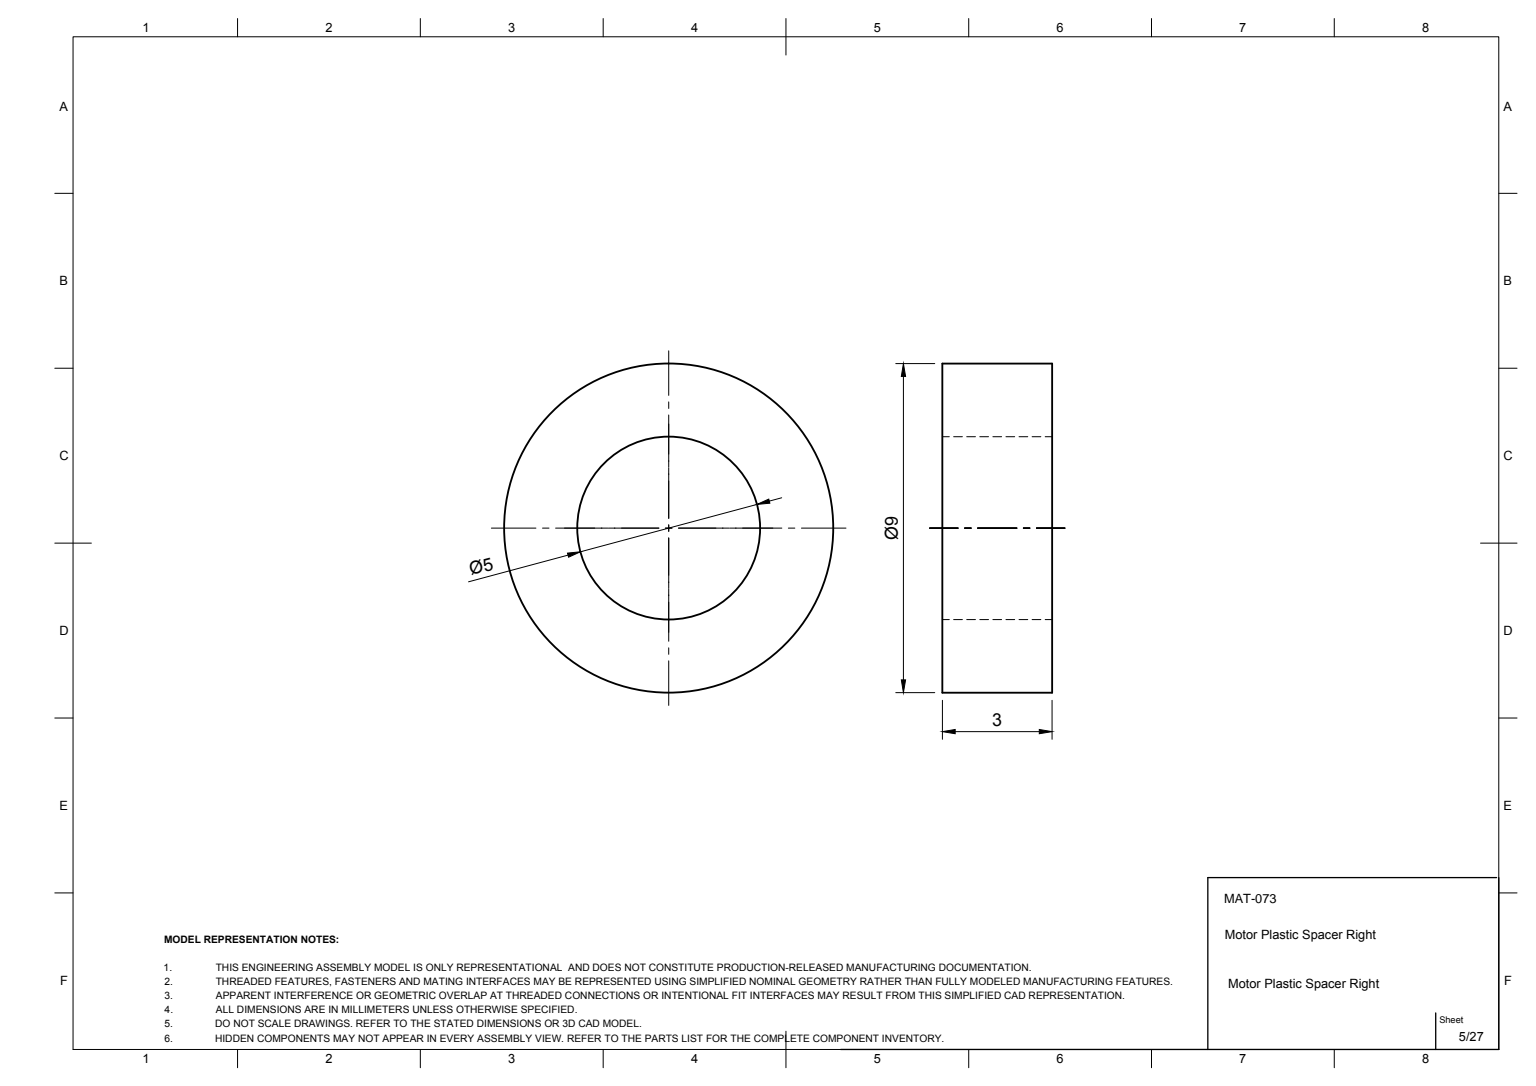
ISO-10303-21;
HEADER;
/* Generated by software containing ST-Developer
 * from STEP Tools, Inc. (www.steptools.com) 
 */

FILE_DESCRIPTION(
/* description */ ('CAx-IF Rec.Pracs.---Representation and Presentation of Product Manufa
cturing Information (PMI)---4.0---2014-10-13'),
/* implementation_level */ '2;1');

FILE_NAME(
/* name */ 'Motor Plastic Spacer Right.step',
/* time_stamp */ '2026-10-24T18:52:33-07:00',
/* author */ (''),
/* organization */ (''),
/* preprocessor_version */ 'ST-DEVELOPER v20.2',
/* originating_system */ 'Autodesk Translation Framework v15.17.0.0',
/* authorisation */ '');

FILE_SCHEMA (('AP242_MANAGED_MODEL_BASED_3D_ENGINEERING_MIM_LF { 1 0 10303 442 2 1 4 }'));
ENDSEC;

DATA;
#10=MECHANICAL_DESIGN_GEOMETRIC_PRESENTATION_REPRESENTATION('',(#416),#34876);
#350=SHAPE_REPRESENTATION_RELATIONSHIP('SRR','None',#34987,#383);
#383=ADVANCED_BREP_SHAPE_REPRESENTATION('',(#449),#34845);
#416=STYLED_ITEM('',(#35161),#449);
#449=MANIFOLD_SOLID_BREP('Motor Plastic Spacer Right',#19556);
#482=FACE_BOUND('',#5883,.T.);
#483=FACE_BOUND('',#5887,.T.);
#606=PLANE('',#20051);
#607=PLANE('',#20058);
#1143=LINE('',#28714,#2742);
#1144=LINE('',#28719,#2743);
#2742=VECTOR('',#22526,0.0025);
#2743=VECTOR('',#22533,0.0045);
#4305=CYLINDRICAL_SURFACE('',#20054,0.0025);
#4306=CYLINDRICAL_SURFACE('',#20056,0.0045);
#4835=FACE_OUTER_BOUND('',#5882,.T.);
#4836=FACE_OUTER_BOUND('',#5884,.T.);
#4837=FACE_OUTER_BOUND('',#5885,.T.);
#4838=FACE_OUTER_BOUND('',#5886,.T.);
#5882=EDGE_LOOP('',(#13034));
#5883=EDGE_LOOP('',(#13035));
#5884=EDGE_LOOP('',(#13036,#13037,#13038,#13039));
#5885=EDGE_LOOP('',(#13040,#13041,#13042,#13043));
#5886=EDGE_LOOP('',(#13044));
#5887=EDGE_LOOP('',(#13045));
#7047=CIRCLE('',#20052,0.00450000000001);
#7048=CIRCLE('',#20053,0.00250000000001);
#7049=CIRCLE('',#20055,0.00250000000001);
#7050=CIRCLE('',#20057,0.00450000000001);
#8149=VERTEX_POINT('',#28708);
#8150=VERTEX_POINT('',#28710);
#8151=VERTEX_POINT('',#28713);
#8152=VERTEX_POINT('',#28717);
#10075=EDGE_CURVE('',#8149,#8149,#7047,.T.);
#10076=EDGE_CURVE('',#8150,#8150,#7048,.T.);
#10077=EDGE_CURVE('',#8150,#8151,#1143,.T.);
#10078=EDGE_CURVE('',#8151,#8151,#7049,.T.);
#10079=EDGE_CURVE('',#8152,#8152,#7050,.T.);
#10080=EDGE_CURVE('',#8152,#8149,#1144,.T.);
#13034=ORIENTED_EDGE('',*,*,#10075,.T.);
#13035=ORIENTED_EDGE('',*,*,#10076,.T.);
#13036=ORIENTED_EDGE('',*,*,#10076,.F.);
#13037=ORIENTED_EDGE('',*,*,#10077,.T.);
#13038=ORIENTED_EDGE('',*,*,#10078,.F.);
#13039=ORIENTED_EDGE('',*,*,#10077,.F.);
#13040=ORIENTED_EDGE('',*,*,#10079,.F.);
#13041=ORIENTED_EDGE('',*,*,#10080,.T.);
#13042=ORIENTED_EDGE('',*,*,#10075,.F.);
#13043=ORIENTED_EDGE('',*,*,#10080,.F.);
#13044=ORIENTED_EDGE('',*,*,#10079,.T.);
#13045=ORIENTED_EDGE('',*,*,#10078,.T.);
#18551=ADVANCED_FACE('',(#4835,#482),#606,.F.);
#18552=ADVANCED_FACE('',(#4836),#4305,.F.);
#18553=ADVANCED_FACE('',(#4837),#4306,.T.);
#18554=ADVANCED_FACE('',(#4838,#483),#607,.T.);
#19556=CLOSED_SHELL('',(#18551,#18552,#18553,#18554));
#20050=AXIS2_PLACEMENT_3D('',#28706,#22516,#22517);
#20051=AXIS2_PLACEMENT_3D('',#28707,#22518,#22519);
#20052=AXIS2_PLACEMENT_3D('',#28709,#22520,#22521);
#20053=AXIS2_PLACEMENT_3D('',#28711,#22522,#22523);
#20054=AXIS2_PLACEMENT_3D('',#28712,#22524,#22525);
#20055=AXIS2_PLACEMENT_3D('',#28715,#22527,#22528);
#20056=AXIS2_PLACEMENT_3D('',#28716,#22529,#22530);
#20057=AXIS2_PLACEMENT_3D('',#28718,#22531,#22532);
#20058=AXIS2_PLACEMENT_3D('',#28720,#22534,#22535);
#22516=DIRECTION('axis',(0.,0.,1.));
#22517=DIRECTION('refdir',(1.,0.,0.));
#22518=DIRECTION('center_axis',(-2.07638679158937E-16,1.,-9.61039042249231E-32));
#22519=DIRECTION('ref_axis',(0.999984788371283,2.07635520636442E-16,-0.00551570721125971));
#22520=DIRECTION('center_axis',(2.07638679158937E-16,-1.,9.61039042249231E-32));
#22521=DIRECTION('ref_axis',(-0.999984788371283,-2.07635520636442E-16,0.00551570721125971));
#22522=DIRECTION('center_axis',(-2.07638679158937E-16,1.,-9.61039042249231E-32));
#22523=DIRECTION('ref_axis',(0.999984788371283,2.07635520636442E-16,-0.00551570721125971));
#22524=DIRECTION('center_axis',(-2.07638679158937E-16,1.,-9.61039042249231E-32));
#22525=DIRECTION('ref_axis',(0.999984788371283,2.07635520636442E-16,-0.00551570721125971));
#22526=DIRECTION('',(-2.07638679158937E-16,1.,-9.61039042249231E-32));
#22527=DIRECTION('center_axis',(2.07638679158937E-16,-1.,9.61039042249231E-32));
#22528=DIRECTION('ref_axis',(0.999984788371283,2.07635520636442E-16,-0.00551570721125971));
#22529=DIRECTION('center_axis',(-2.07638679158937E-16,1.,-9.61039042249231E-32));
#22530=DIRECTION('ref_axis',(-0.999984788371283,-2.07635520636442E-16,0.00551570721125971));
#22531=DIRECTION('center_axis',(-2.07638679158937E-16,1.,-9.61039042249231E-32));
#22532=DIRECTION('ref_axis',(-0.999984788371283,-2.07635520636442E-16,0.00551570721125971));
#22533=DIRECTION('',(2.07638679158937E-16,-1.,9.61039042249231E-32));
#22534=DIRECTION('center_axis',(-2.07638679158937E-16,1.,-9.61039042249231E-32));
#22535=DIRECTION('ref_axis',(0.999984788371283,2.07635520636442E-16,-0.00551570721125971));
#28706=CARTESIAN_POINT('',(0.,0.,0.));
#28707=CARTESIAN_POINT('Origin',(-4.36800060759181E-17,-0.02565,1.40756589985541E-33));
#28708=CARTESIAN_POINT('',(0.00449993154767073,-0.02565000000001,-2.48206824506692E-5));
#28709=CARTESIAN_POINT('Origin',(-4.3680006075916E-17,-0.02565000000001,
1.40756589985638E-33));
#28710=CARTESIAN_POINT('',(-0.00249996197092825,-0.02565000000001,1.37892680281496E-5));
#28711=CARTESIAN_POINT('Origin',(-4.3680006075916E-17,-0.02565000000001,
1.40756589985638E-33));
#28712=CARTESIAN_POINT('Origin',(-4.39914640946565E-17,-0.02415,1.26341004351803E-33));
#28713=CARTESIAN_POINT('',(-0.00249996197092825,-0.02264999999999,1.37892680281496E-5));
#28714=CARTESIAN_POINT('',(-0.00249996197092825,-0.02415,1.37892680281496E-5));
#28715=CARTESIAN_POINT('Origin',(-4.4302922113397E-17,-0.02264999999999,
1.11925418717968E-33));
#28716=CARTESIAN_POINT('Origin',(-4.39914640946565E-17,-0.02415,1.26341004351803E-33));
#28717=CARTESIAN_POINT('',(0.00449993154767073,-0.02264999999999,-2.48206824506692E-5));
#28718=CARTESIAN_POINT('Origin',(-4.4302922113397E-17,-0.02264999999999,
1.11925418717968E-33));
#28719=CARTESIAN_POINT('',(0.00449993154767073,-0.02415,-2.48206824506692E-5));
#28720=CARTESIAN_POINT('Origin',(-4.43029221133949E-17,-0.02265,1.11925418718065E-33));
#34810=UNCERTAINTY_MEASURE_WITH_UNIT(LENGTH_MEASURE(1.E-5),#34877,
'DISTANCE_ACCURACY_VALUE',
'Maximum model space distance between geometric entities at asserted c
onnectivities');
#34841=UNCERTAINTY_MEASURE_WITH_UNIT(LENGTH_MEASURE(1.E-5),#34877,
'DISTANCE_ACCURACY_VALUE',
'Maximum model space distance between geometric entities at asserted c
onnectivities');
#34845=(
GEOMETRIC_REPRESENTATION_CONTEXT(3)
GLOBAL_UNCERTAINTY_ASSIGNED_CONTEXT((#34810))
GLOBAL_UNIT_ASSIGNED_CONTEXT((#34877,#34878,#34879))
REPRESENTATION_CONTEXT('','3D')
);
#34876=(
GEOMETRIC_REPRESENTATION_CONTEXT(3)
GLOBAL_UNCERTAINTY_ASSIGNED_CONTEXT((#34841))
GLOBAL_UNIT_ASSIGNED_CONTEXT((#34877,#34878,#34879))
REPRESENTATION_CONTEXT('','3D')
);
#34877=(
LENGTH_UNIT()
NAMED_UNIT(*)
SI_UNIT($,.METRE.)
);
#34878=(
NAMED_UNIT(*)
PLANE_ANGLE_UNIT()
SI_UNIT($,.RADIAN.)
);
#34879=(
NAMED_UNIT(*)
SI_UNIT($,.STERADIAN.)
SOLID_ANGLE_UNIT()
);
#34883=SHAPE_DEFINITION_REPRESENTATION(#34917,#34987);
#34917=PRODUCT_DEFINITION_SHAPE('',$,#35022);
#34987=SHAPE_REPRESENTATION('',(#20050),#34845);
#35018=PRODUCT_DEFINITION_CONTEXT('part definition',#35122,'design');
#35022=PRODUCT_DEFINITION('Motor Plastic Spacer Right',
'Motor Plastic Spacer Right',#35056,#35018);
#35056=PRODUCT_DEFINITION_FORMATION('',$,#35127);
#35122=APPLICATION_CONTEXT('Managed model based 3d engineering');
#35123=PRODUCT_CONTEXT('part definition',#35122,'mechanical');
#35127=PRODUCT('Motor Plastic Spacer Right',
'Motor Plastic Spacer Right',
'LEGAL AND USAGE DISCLAIMER: this Data/Model is provided \X2\201C\X0\A
S IS\X2\201D\X0\ for informational and representational only. It is a 
geometric approximation and is NOT engineered, certified, or guarantee
d for dimensional accuracy, exact tolerances, or production-level prec
ision. Vendor disclaims all implied warranties including fitness for a
 particular purpose. DO NOT USE FOR DIRECT PHYSICAL MANUFACTURING, AUT
OMATED PRODUCTION, OR SAFETY-CRITICAL SYSTEMS without independent engi
neering verification and resolution of any design discrepancies.',(#35123));
#35161=PRESENTATION_STYLE_ASSIGNMENT((#35170));
#35170=SURFACE_STYLE_USAGE(.BOTH.,#35179);
#35179=SURFACE_SIDE_STYLE('',(#35188));
#35188=SURFACE_STYLE_FILL_AREA(#35197);
#35197=FILL_AREA_STYLE('Aluminum - Anodized Glossy (Blue)',(#35206));
#35206=FILL_AREA_STYLE_COLOUR('Aluminum - Anodized Glossy (Blue)',#35215);
#35215=COLOUR_RGB('Aluminum - Anodized Glossy (Blue)',0.349019607843137,
0.584313725490196,0.854901960784314);
ENDSEC;
END-ISO-10303-21;
